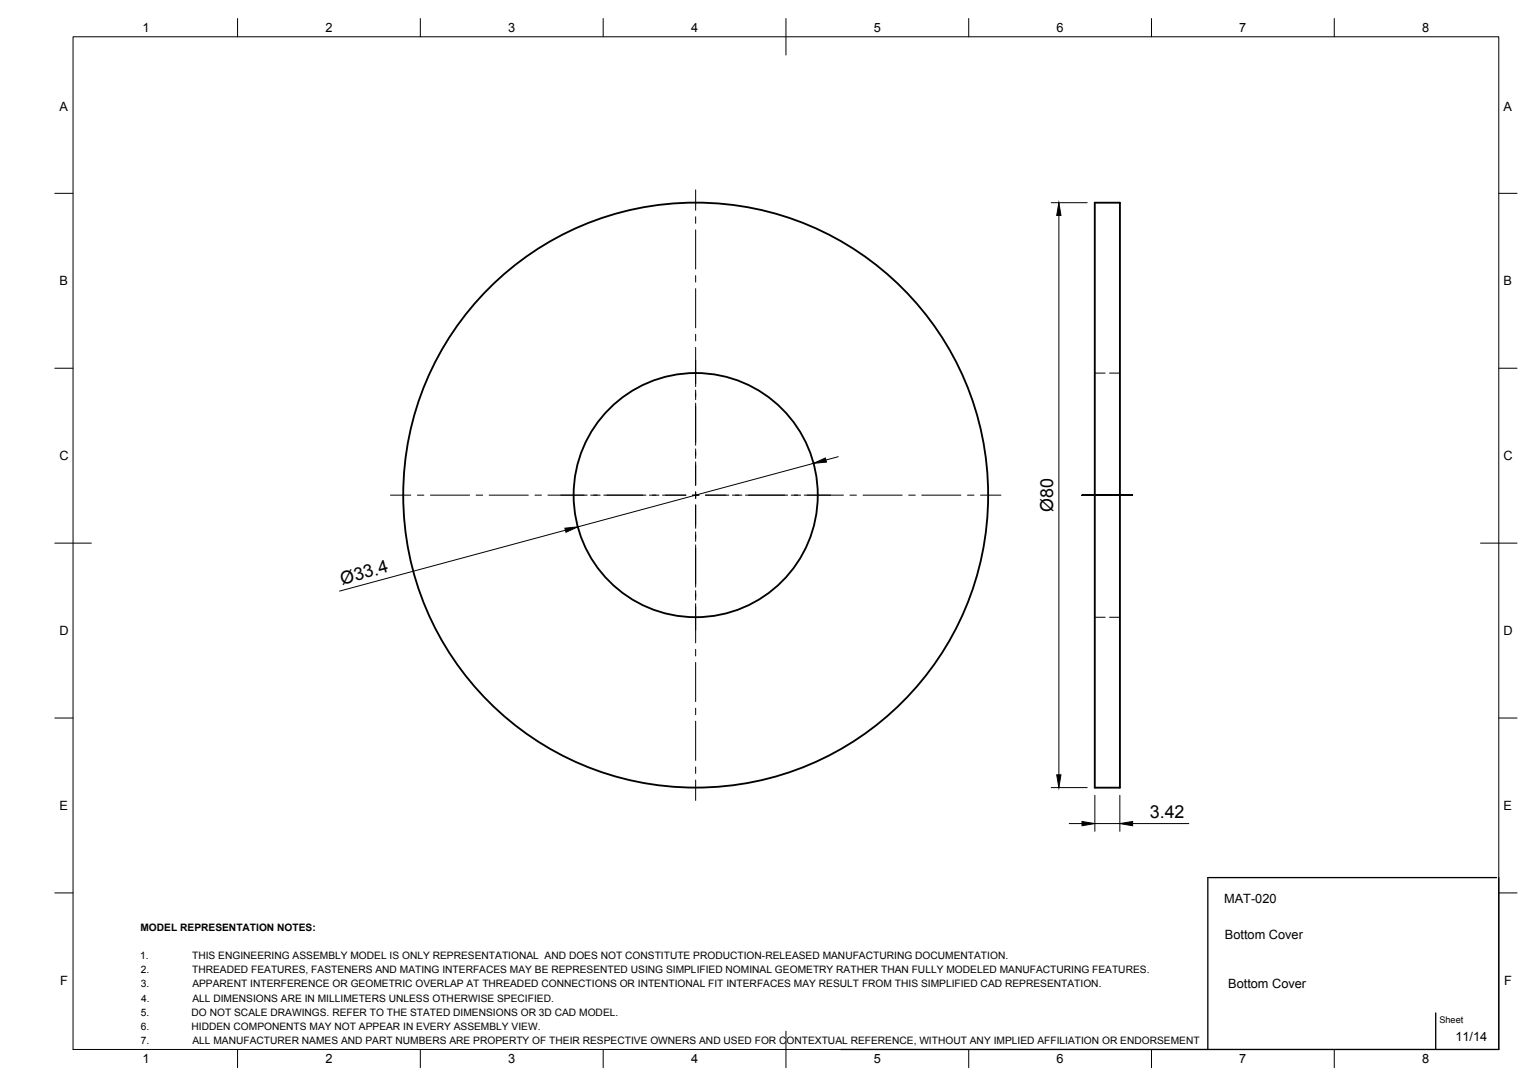
ISO-10303-21;
HEADER;
/* Generated by software containing ST-Developer
 * from STEP Tools, Inc. (www.steptools.com) 
 */

FILE_DESCRIPTION(
/* description */ ('STEP AP214'),
/* implementation_level */ '2;1');

FILE_NAME(
/* name */ 'Bottom Cover.step',
/* time_stamp */ '2026-11-14T06:20:50-08:00',
/* author */ (''),
/* organization */ (''),
/* preprocessor_version */ 'ST-DEVELOPER v20.2',
/* originating_system */ 'Autodesk Translation Framework v15.17.0.0',
/* authorisation */ '');

FILE_SCHEMA (('AUTOMOTIVE_DESIGN { 1 0 10303 214 3 1 1 }'));
ENDSEC;

DATA;
#10=MECHANICAL_DESIGN_GEOMETRIC_PRESENTATION_REPRESENTATION('',(#962),#20658);
#132=FACE_BOUND('',#1349,.T.);
#133=FACE_BOUND('',#1351,.T.);
#424=PLANE('',#3979);
#425=PLANE('',#3980);
#593=LINE('',#20313,#786);
#594=LINE('',#20319,#787);
#786=VECTOR('',#4632,16.7);
#787=VECTOR('',#4639,40.);
#906=CYLINDRICAL_SURFACE('',#3973,16.7);
#907=CYLINDRICAL_SURFACE('',#3976,40.);
#938=SHAPE_REPRESENTATION_RELATIONSHIP('SRR','None',#20722,#950);
#950=ADVANCED_BREP_SHAPE_REPRESENTATION('',(#974),#20652);
#962=STYLED_ITEM('',(#20785),#974);
#974=MANIFOLD_SOLID_BREP('Body1',#3657);
#1129=FACE_OUTER_BOUND('',#1346,.T.);
#1130=FACE_OUTER_BOUND('',#1347,.T.);
#1131=FACE_OUTER_BOUND('',#1348,.T.);
#1132=FACE_OUTER_BOUND('',#1350,.T.);
#1346=EDGE_LOOP('',(#3206,#3207,#3208,#3209));
#1347=EDGE_LOOP('',(#3210,#3211,#3212,#3213));
#1348=EDGE_LOOP('',(#3214));
#1349=EDGE_LOOP('',(#3215));
#1350=EDGE_LOOP('',(#3216));
#1351=EDGE_LOOP('',(#3217));
#1485=CIRCLE('',#3974,16.7);
#1486=CIRCLE('',#3975,16.7);
#1487=CIRCLE('',#3977,40.);
#1488=CIRCLE('',#3978,40.);
#1813=VERTEX_POINT('',#20310);
#1814=VERTEX_POINT('',#20312);
#1815=VERTEX_POINT('',#20316);
#1816=VERTEX_POINT('',#20318);
#2285=EDGE_CURVE('',#1813,#1813,#1485,.T.);
#2286=EDGE_CURVE('',#1813,#1814,#593,.T.);
#2287=EDGE_CURVE('',#1814,#1814,#1486,.T.);
#2288=EDGE_CURVE('',#1815,#1815,#1487,.T.);
#2289=EDGE_CURVE('',#1815,#1816,#594,.T.);
#2290=EDGE_CURVE('',#1816,#1816,#1488,.T.);
#3206=ORIENTED_EDGE('',*,*,#2285,.T.);
#3207=ORIENTED_EDGE('',*,*,#2286,.T.);
#3208=ORIENTED_EDGE('',*,*,#2287,.F.);
#3209=ORIENTED_EDGE('',*,*,#2286,.F.);
#3210=ORIENTED_EDGE('',*,*,#2288,.T.);
#3211=ORIENTED_EDGE('',*,*,#2289,.T.);
#3212=ORIENTED_EDGE('',*,*,#2290,.F.);
#3213=ORIENTED_EDGE('',*,*,#2289,.F.);
#3214=ORIENTED_EDGE('',*,*,#2290,.T.);
#3215=ORIENTED_EDGE('',*,*,#2285,.F.);
#3216=ORIENTED_EDGE('',*,*,#2288,.F.);
#3217=ORIENTED_EDGE('',*,*,#2287,.T.);
#3591=ADVANCED_FACE('',(#1129),#906,.F.);
#3592=ADVANCED_FACE('',(#1130),#907,.T.);
#3593=ADVANCED_FACE('',(#1131,#132),#424,.T.);
#3594=ADVANCED_FACE('',(#1132,#133),#425,.F.);
#3657=CLOSED_SHELL('',(#3591,#3592,#3593,#3594));
#3972=AXIS2_PLACEMENT_3D('',#20308,#4626,#4627);
#3973=AXIS2_PLACEMENT_3D('',#20309,#4628,#4629);
#3974=AXIS2_PLACEMENT_3D('',#20311,#4630,#4631);
#3975=AXIS2_PLACEMENT_3D('',#20314,#4633,#4634);
#3976=AXIS2_PLACEMENT_3D('',#20315,#4635,#4636);
#3977=AXIS2_PLACEMENT_3D('',#20317,#4637,#4638);
#3978=AXIS2_PLACEMENT_3D('',#20320,#4640,#4641);
#3979=AXIS2_PLACEMENT_3D('',#20321,#4642,#4643);
#3980=AXIS2_PLACEMENT_3D('',#20322,#4644,#4645);
#4626=DIRECTION('axis',(0.,0.,1.));
#4627=DIRECTION('refdir',(1.,0.,0.));
#4628=DIRECTION('center_axis',(0.,0.,-1.));
#4629=DIRECTION('ref_axis',(-1.,0.,0.));
#4630=DIRECTION('center_axis',(0.,0.,1.));
#4631=DIRECTION('ref_axis',(1.,0.,0.));
#4632=DIRECTION('',(0.,0.,-1.));
#4633=DIRECTION('center_axis',(0.,0.,1.));
#4634=DIRECTION('ref_axis',(1.,0.,0.));
#4635=DIRECTION('center_axis',(0.,0.,-1.));
#4636=DIRECTION('ref_axis',(-1.,0.,0.));
#4637=DIRECTION('center_axis',(0.,0.,1.));
#4638=DIRECTION('ref_axis',(1.,0.,0.));
#4639=DIRECTION('',(0.,0.,1.));
#4640=DIRECTION('center_axis',(0.,0.,1.));
#4641=DIRECTION('ref_axis',(1.,0.,0.));
#4642=DIRECTION('center_axis',(0.,0.,1.));
#4643=DIRECTION('ref_axis',(1.,0.,0.));
#4644=DIRECTION('center_axis',(0.,0.,1.));
#4645=DIRECTION('ref_axis',(1.,0.,0.));
#20308=CARTESIAN_POINT('',(0.,0.,0.));
#20309=CARTESIAN_POINT('Origin',(0.,0.,3.42));
#20310=CARTESIAN_POINT('',(16.7,-2.04516015457608E-15,3.42));
#20311=CARTESIAN_POINT('Origin',(0.,0.,3.42));
#20312=CARTESIAN_POINT('',(16.7,-2.04516015457608E-15,0.));
#20313=CARTESIAN_POINT('',(16.7,-2.04516015457608E-15,3.42));
#20314=CARTESIAN_POINT('Origin',(0.,0.,0.));
#20315=CARTESIAN_POINT('Origin',(0.,0.,3.42));
#20316=CARTESIAN_POINT('',(40.,-4.89858719658941E-15,0.));
#20317=CARTESIAN_POINT('Origin',(0.,0.,0.));
#20318=CARTESIAN_POINT('',(40.,-4.89858719658941E-15,3.42));
#20319=CARTESIAN_POINT('',(40.,-4.89858719658941E-15,3.42));
#20320=CARTESIAN_POINT('Origin',(0.,0.,3.42));
#20321=CARTESIAN_POINT('Origin',(0.,0.,3.42));
#20322=CARTESIAN_POINT('Origin',(0.,0.,0.));
#20638=UNCERTAINTY_MEASURE_WITH_UNIT(LENGTH_MEASURE(0.01),#20659,
'DISTANCE_ACCURACY_VALUE',
'Maximum model space distance between geometric entities at asserted c
onnectivities');
#20644=UNCERTAINTY_MEASURE_WITH_UNIT(LENGTH_MEASURE(0.01),#20659,
'DISTANCE_ACCURACY_VALUE',
'Maximum model space distance between geometric entities at asserted c
onnectivities');
#20652=(
GEOMETRIC_REPRESENTATION_CONTEXT(3)
GLOBAL_UNCERTAINTY_ASSIGNED_CONTEXT((#20638))
GLOBAL_UNIT_ASSIGNED_CONTEXT((#20659,#20661,#20662))
REPRESENTATION_CONTEXT('','3D')
);
#20658=(
GEOMETRIC_REPRESENTATION_CONTEXT(3)
GLOBAL_UNCERTAINTY_ASSIGNED_CONTEXT((#20644))
GLOBAL_UNIT_ASSIGNED_CONTEXT((#20659,#20661,#20662))
REPRESENTATION_CONTEXT('','3D')
);
#20659=(
LENGTH_UNIT()
NAMED_UNIT(*)
SI_UNIT(.MILLI.,.METRE.)
);
#20661=(
NAMED_UNIT(*)
PLANE_ANGLE_UNIT()
SI_UNIT($,.RADIAN.)
);
#20662=(
NAMED_UNIT(*)
SI_UNIT($,.STERADIAN.)
SOLID_ANGLE_UNIT()
);
#20670=SHAPE_DEFINITION_REPRESENTATION(#20683,#20722);
#20683=PRODUCT_DEFINITION_SHAPE('',$,#20736);
#20722=SHAPE_REPRESENTATION('',(#3972),#20652);
#20728=PRODUCT_DEFINITION_CONTEXT('part definition',#20769,'design');
#20736=PRODUCT_DEFINITION('Bottom Cover','Bottom Cover',#20749,#20728);
#20749=PRODUCT_DEFINITION_FORMATION('',$,#20778);
#20769=APPLICATION_CONTEXT(
'Core Data for Automotive Mechanical Design Process');
#20770=PRODUCT_CONTEXT('part definition',#20769,'mechanical');
#20778=PRODUCT('Bottom Cover','Bottom Cover',$,(#20770));
#20785=PRESENTATION_STYLE_ASSIGNMENT((#20790));
#20790=SURFACE_STYLE_USAGE(.BOTH.,#20795);
#20795=SURFACE_SIDE_STYLE('',(#20800));
#20800=SURFACE_STYLE_FILL_AREA(#20805);
#20805=FILL_AREA_STYLE('Opaque(97,158,199)',(#20810));
#20810=FILL_AREA_STYLE_COLOUR('Opaque(97,158,199)',#20815);
#20815=COLOUR_RGB('Opaque(97,158,199)',0.380392156862745,0.619607843137255,
0.780392156862745);
ENDSEC;
END-ISO-10303-21;
